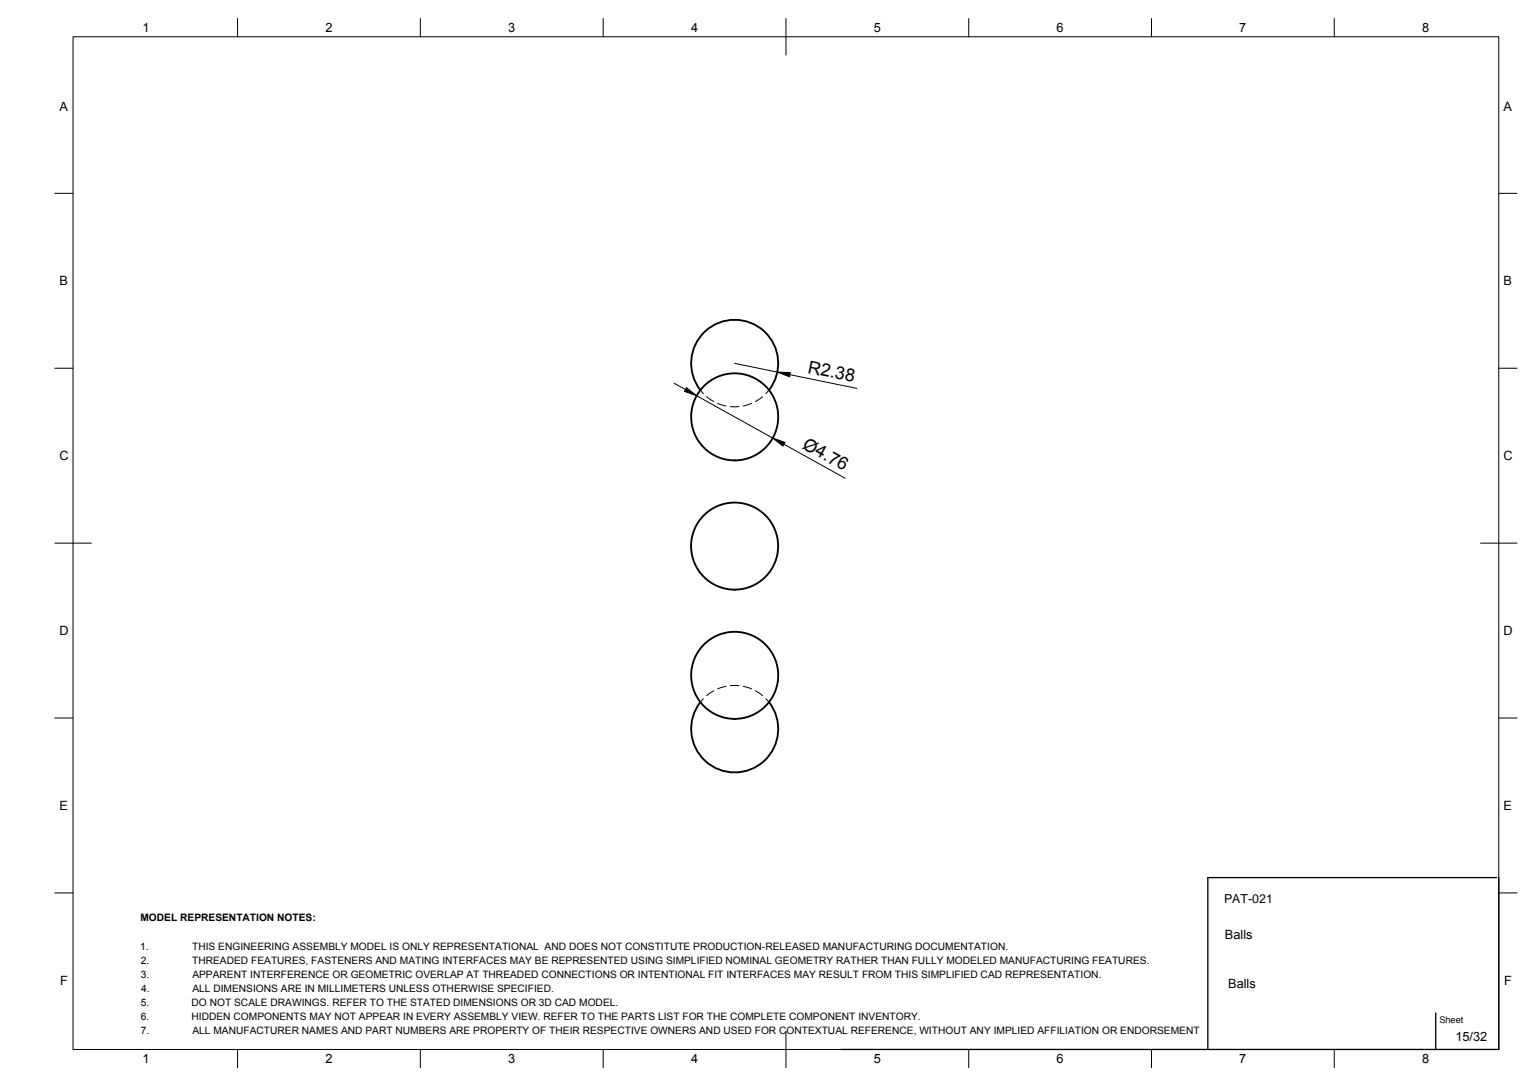
ISO-10303-21;
HEADER;
/* Generated by software containing ST-Developer
 * from STEP Tools, Inc. (www.steptools.com) 
 */

FILE_DESCRIPTION(
/* description */ ('Chain-less indexing wheel (Geneva) drive'),
/* implementation_level */ '2;1');

FILE_NAME(
/* name */ 'Balls.step',
/* time_stamp */ '2026-10-28T03:25:22-07:00',
/* author */ (''),
/* organization */ (''),
/* preprocessor_version */ 'ST-DEVELOPER v20.2',
/* originating_system */ 'Autodesk Translation Framework v15.17.0.0',
/* authorisation */ '');

FILE_SCHEMA (('AUTOMOTIVE_DESIGN { 1 0 10303 214 3 1 1 }'));
ENDSEC;

DATA;
#10=MECHANICAL_DESIGN_GEOMETRIC_PRESENTATION_REPRESENTATION('',(#312,#313,#314,#315,#316,#317,#318,#319),#10957);
#179=SPHERICAL_SURFACE('',#6312,0.23815);
#180=SPHERICAL_SURFACE('',#6314,0.23815);
#181=SPHERICAL_SURFACE('',#6316,0.23815);
#182=SPHERICAL_SURFACE('',#6318,0.23815);
#183=SPHERICAL_SURFACE('',#6320,0.23815);
#184=SPHERICAL_SURFACE('',#6322,0.23815);
#185=SPHERICAL_SURFACE('',#6324,0.23815);
#186=SPHERICAL_SURFACE('',#6326,0.23815);
#262=SHAPE_REPRESENTATION_RELATIONSHIP('SRR','None',#11076,#287);
#287=ADVANCED_BREP_SHAPE_REPRESENTATION('',(#344,#345,#346,#347,#348,#349,
#350,#351),#10939);
#312=STYLED_ITEM('',(#11287),#344);
#313=STYLED_ITEM('',(#11287),#345);
#314=STYLED_ITEM('',(#11287),#346);
#315=STYLED_ITEM('',(#11287),#347);
#316=STYLED_ITEM('',(#11287),#348);
#317=STYLED_ITEM('',(#11287),#349);
#318=STYLED_ITEM('',(#11287),#350);
#319=STYLED_ITEM('',(#11287),#351);
#344=MANIFOLD_SOLID_BREP('Body1',#5709);
#345=MANIFOLD_SOLID_BREP('Body2',#5710);
#346=MANIFOLD_SOLID_BREP('Body3',#5711);
#347=MANIFOLD_SOLID_BREP('Body4',#5712);
#348=MANIFOLD_SOLID_BREP('Body5',#5713);
#349=MANIFOLD_SOLID_BREP('Body6',#5714);
#350=MANIFOLD_SOLID_BREP('Body7',#5715);
#351=MANIFOLD_SOLID_BREP('Body8',#5716);
#793=FACE_OUTER_BOUND('',#1187,.T.);
#794=FACE_OUTER_BOUND('',#1188,.T.);
#795=FACE_OUTER_BOUND('',#1189,.T.);
#796=FACE_OUTER_BOUND('',#1190,.T.);
#797=FACE_OUTER_BOUND('',#1191,.T.);
#798=FACE_OUTER_BOUND('',#1192,.T.);
#799=FACE_OUTER_BOUND('',#1193,.T.);
#800=FACE_OUTER_BOUND('',#1194,.T.);
#1187=EDGE_LOOP('',(#4363,#4364));
#1188=EDGE_LOOP('',(#4365,#4366));
#1189=EDGE_LOOP('',(#4367,#4368));
#1190=EDGE_LOOP('',(#4369,#4370));
#1191=EDGE_LOOP('',(#4371,#4372));
#1192=EDGE_LOOP('',(#4373,#4374));
#1193=EDGE_LOOP('',(#4375,#4376));
#1194=EDGE_LOOP('',(#4377,#4378));
#2319=CIRCLE('',#6313,0.23815);
#2320=CIRCLE('',#6315,0.23815);
#2321=CIRCLE('',#6317,0.23815);
#2322=CIRCLE('',#6319,0.23815);
#2323=CIRCLE('',#6321,0.23815);
#2324=CIRCLE('',#6323,0.23815);
#2325=CIRCLE('',#6325,0.23815);
#2326=CIRCLE('',#6327,0.23815);
#2697=VERTEX_POINT('',#9322);
#2698=VERTEX_POINT('',#9323);
#2699=VERTEX_POINT('',#9326);
#2700=VERTEX_POINT('',#9327);
#2701=VERTEX_POINT('',#9330);
#2702=VERTEX_POINT('',#9331);
#2703=VERTEX_POINT('',#9334);
#2704=VERTEX_POINT('',#9335);
#2705=VERTEX_POINT('',#9338);
#2706=VERTEX_POINT('',#9339);
#2707=VERTEX_POINT('',#9342);
#2708=VERTEX_POINT('',#9343);
#2709=VERTEX_POINT('',#9346);
#2710=VERTEX_POINT('',#9347);
#2711=VERTEX_POINT('',#9350);
#2712=VERTEX_POINT('',#9351);
#3307=EDGE_CURVE('',#2697,#2698,#2319,.T.);
#3308=EDGE_CURVE('',#2699,#2700,#2320,.T.);
#3309=EDGE_CURVE('',#2701,#2702,#2321,.T.);
#3310=EDGE_CURVE('',#2703,#2704,#2322,.T.);
#3311=EDGE_CURVE('',#2705,#2706,#2323,.T.);
#3312=EDGE_CURVE('',#2707,#2708,#2324,.T.);
#3313=EDGE_CURVE('',#2709,#2710,#2325,.T.);
#3314=EDGE_CURVE('',#2711,#2712,#2326,.T.);
#4363=ORIENTED_EDGE('',*,*,#3307,.T.);
#4364=ORIENTED_EDGE('',*,*,#3307,.F.);
#4365=ORIENTED_EDGE('',*,*,#3308,.T.);
#4366=ORIENTED_EDGE('',*,*,#3308,.F.);
#4367=ORIENTED_EDGE('',*,*,#3309,.T.);
#4368=ORIENTED_EDGE('',*,*,#3309,.F.);
#4369=ORIENTED_EDGE('',*,*,#3310,.T.);
#4370=ORIENTED_EDGE('',*,*,#3310,.F.);
#4371=ORIENTED_EDGE('',*,*,#3311,.T.);
#4372=ORIENTED_EDGE('',*,*,#3311,.F.);
#4373=ORIENTED_EDGE('',*,*,#3312,.T.);
#4374=ORIENTED_EDGE('',*,*,#3312,.F.);
#4375=ORIENTED_EDGE('',*,*,#3313,.T.);
#4376=ORIENTED_EDGE('',*,*,#3313,.F.);
#4377=ORIENTED_EDGE('',*,*,#3314,.T.);
#4378=ORIENTED_EDGE('',*,*,#3314,.F.);
#5507=ADVANCED_FACE('',(#793),#179,.T.);
#5508=ADVANCED_FACE('',(#794),#180,.T.);
#5509=ADVANCED_FACE('',(#795),#181,.T.);
#5510=ADVANCED_FACE('',(#796),#182,.T.);
#5511=ADVANCED_FACE('',(#797),#183,.T.);
#5512=ADVANCED_FACE('',(#798),#184,.T.);
#5513=ADVANCED_FACE('',(#799),#185,.T.);
#5514=ADVANCED_FACE('',(#800),#186,.T.);
#5709=CLOSED_SHELL('',(#5507));
#5710=CLOSED_SHELL('',(#5508));
#5711=CLOSED_SHELL('',(#5509));
#5712=CLOSED_SHELL('',(#5510));
#5713=CLOSED_SHELL('',(#5511));
#5714=CLOSED_SHELL('',(#5512));
#5715=CLOSED_SHELL('',(#5513));
#5716=CLOSED_SHELL('',(#5514));
#6311=AXIS2_PLACEMENT_3D('',#9320,#7509,#7510);
#6312=AXIS2_PLACEMENT_3D('',#9321,#7511,#7512);
#6313=AXIS2_PLACEMENT_3D('',#9324,#7513,#7514);
#6314=AXIS2_PLACEMENT_3D('',#9325,#7515,#7516);
#6315=AXIS2_PLACEMENT_3D('',#9328,#7517,#7518);
#6316=AXIS2_PLACEMENT_3D('',#9329,#7519,#7520);
#6317=AXIS2_PLACEMENT_3D('',#9332,#7521,#7522);
#6318=AXIS2_PLACEMENT_3D('',#9333,#7523,#7524);
#6319=AXIS2_PLACEMENT_3D('',#9336,#7525,#7526);
#6320=AXIS2_PLACEMENT_3D('',#9337,#7527,#7528);
#6321=AXIS2_PLACEMENT_3D('',#9340,#7529,#7530);
#6322=AXIS2_PLACEMENT_3D('',#9341,#7531,#7532);
#6323=AXIS2_PLACEMENT_3D('',#9344,#7533,#7534);
#6324=AXIS2_PLACEMENT_3D('',#9345,#7535,#7536);
#6325=AXIS2_PLACEMENT_3D('',#9348,#7537,#7538);
#6326=AXIS2_PLACEMENT_3D('',#9349,#7539,#7540);
#6327=AXIS2_PLACEMENT_3D('',#9352,#7541,#7542);
#7509=DIRECTION('axis',(0.,0.,1.));
#7510=DIRECTION('refdir',(1.,0.,0.));
#7511=DIRECTION('center_axis',(0.,0.,1.));
#7512=DIRECTION('ref_axis',(1.,0.,0.));
#7513=DIRECTION('center_axis',(1.22464679914735E-16,-1.,0.));
#7514=DIRECTION('ref_axis',(-1.,-1.22464679914735E-16,0.));
#7515=DIRECTION('center_axis',(0.707106781186548,0.,0.707106781186548));
#7516=DIRECTION('ref_axis',(0.707106781186548,0.,-0.707106781186548));
#7517=DIRECTION('center_axis',(8.65956056235494E-17,-1.,-8.65956056235493E-17));
#7518=DIRECTION('ref_axis',(-0.707106781186547,-1.22464679914735E-16,0.707106781186547));
#7519=DIRECTION('center_axis',(1.,0.,0.));
#7520=DIRECTION('ref_axis',(6.12323399573676E-17,0.,-1.));
#7521=DIRECTION('center_axis',(7.49879891330929E-33,-1.,-1.22464679914735E-16));
#7522=DIRECTION('ref_axis',(-6.12323399573676E-17,-1.22464679914735E-16,
1.));
#7523=DIRECTION('center_axis',(0.707106781186548,0.,-0.707106781186548));
#7524=DIRECTION('ref_axis',(-0.707106781186548,0.,-0.707106781186548));
#7525=DIRECTION('center_axis',(-8.65956056235493E-17,-1.,-8.65956056235494E-17));
#7526=DIRECTION('ref_axis',(0.707106781186547,-1.22464679914735E-16,0.707106781186547));
#7527=DIRECTION('center_axis',(0.,0.,-1.));
#7528=DIRECTION('ref_axis',(-1.,0.,-1.22464679914735E-16));
#7529=DIRECTION('center_axis',(-1.22464679914735E-16,-1.,-1.49975978266186E-32));
#7530=DIRECTION('ref_axis',(1.,-1.22464679914735E-16,1.22464679914735E-16));
#7531=DIRECTION('center_axis',(-0.707106781186547,0.,-0.707106781186548));
#7532=DIRECTION('ref_axis',(-0.707106781186548,0.,0.707106781186547));
#7533=DIRECTION('center_axis',(-8.65956056235493E-17,-1.,8.65956056235493E-17));
#7534=DIRECTION('ref_axis',(0.707106781186548,-1.22464679914735E-16,-0.707106781186547));
#7535=DIRECTION('center_axis',(-1.,0.,0.));
#7536=DIRECTION('ref_axis',(-1.83697019872103E-16,0.,1.));
#7537=DIRECTION('center_axis',(-2.24963967399279E-32,-1.,1.22464679914735E-16));
#7538=DIRECTION('ref_axis',(1.83697019872103E-16,-1.22464679914735E-16,
-1.));
#7539=DIRECTION('center_axis',(-0.707106781186548,0.,0.707106781186548));
#7540=DIRECTION('ref_axis',(0.707106781186547,0.,0.707106781186548));
#7541=DIRECTION('center_axis',(8.65956056235493E-17,-1.,8.65956056235493E-17));
#7542=DIRECTION('ref_axis',(-0.707106781186547,-1.22464679914735E-16,-0.707106781186548));
#9320=CARTESIAN_POINT('',(0.,0.,0.));
#9321=CARTESIAN_POINT('Origin',(1.,0.,0.));
#9322=CARTESIAN_POINT('',(1.,-1.78583896120461E-33,0.23815));
#9323=CARTESIAN_POINT('',(1.,-1.78583896120461E-33,-0.23815));
#9324=CARTESIAN_POINT('Origin',(1.,0.,0.));
#9325=CARTESIAN_POINT('Origin',(0.707106781186548,0.,-0.707106781186547));
#9326=CARTESIAN_POINT('',(0.875504261126124,-1.78583896120461E-33,-0.538709301246971));
#9327=CARTESIAN_POINT('',(0.538709301246971,-1.78583896120461E-33,-0.875504261126124));
#9328=CARTESIAN_POINT('Origin',(0.707106781186548,0.,-0.707106781186547));
#9329=CARTESIAN_POINT('Origin',(6.12323399573677E-17,0.,-1.));
#9330=CARTESIAN_POINT('',(0.23815,-1.78583896120461E-33,-1.));
#9331=CARTESIAN_POINT('',(-0.23815,-1.78583896120461E-33,-1.));
#9332=CARTESIAN_POINT('Origin',(6.12323399573677E-17,0.,-1.));
#9333=CARTESIAN_POINT('Origin',(-0.707106781186547,0.,-0.707106781186548));
#9334=CARTESIAN_POINT('',(-0.538709301246971,-1.78583896120461E-33,-0.875504261126124));
#9335=CARTESIAN_POINT('',(-0.875504261126124,-1.78583896120461E-33,-0.538709301246971));
#9336=CARTESIAN_POINT('Origin',(-0.707106781186547,0.,-0.707106781186548));
#9337=CARTESIAN_POINT('Origin',(-1.,0.,-1.22464679914735E-16));
#9338=CARTESIAN_POINT('',(-1.,-1.78583896120461E-33,-0.23815));
#9339=CARTESIAN_POINT('',(-1.,-1.78583896120461E-33,0.23815));
#9340=CARTESIAN_POINT('Origin',(-1.,0.,-1.22464679914735E-16));
#9341=CARTESIAN_POINT('Origin',(-0.707106781186548,0.,0.707106781186547));
#9342=CARTESIAN_POINT('',(-0.875504261126124,-7.94881478324376E-33,0.538709301246971));
#9343=CARTESIAN_POINT('',(-0.538709301246971,4.37713686083455E-33,0.875504261126124));
#9344=CARTESIAN_POINT('Origin',(-0.707106781186548,0.,0.707106781186547));
#9345=CARTESIAN_POINT('Origin',(-1.83697019872103E-16,0.,1.));
#9346=CARTESIAN_POINT('',(-0.23815,-1.78583896120461E-33,1.));
#9347=CARTESIAN_POINT('',(0.23815,-1.78583896120461E-33,1.));
#9348=CARTESIAN_POINT('Origin',(-1.83697019872103E-16,0.,1.));
#9349=CARTESIAN_POINT('Origin',(0.707106781186547,0.,0.707106781186548));
#9350=CARTESIAN_POINT('',(0.538709301246971,-4.86732687222419E-33,0.875504261126124));
#9351=CARTESIAN_POINT('',(0.875504261126124,1.29564894981497E-33,0.538709301246971));
#9352=CARTESIAN_POINT('Origin',(0.707106781186547,0.,0.707106781186548));
#10908=UNCERTAINTY_MEASURE_WITH_UNIT(LENGTH_MEASURE(0.001),#10958,
'DISTANCE_ACCURACY_VALUE',
'Maximum model space distance between geometric entities at asserted c
onnectivities');
#10926=UNCERTAINTY_MEASURE_WITH_UNIT(LENGTH_MEASURE(0.001),#10958,
'DISTANCE_ACCURACY_VALUE',
'Maximum model space distance between geometric entities at asserted c
onnectivities');
#10939=(
GEOMETRIC_REPRESENTATION_CONTEXT(3)
GLOBAL_UNCERTAINTY_ASSIGNED_CONTEXT((#10908))
GLOBAL_UNIT_ASSIGNED_CONTEXT((#10958,#10960,#10961))
REPRESENTATION_CONTEXT('','3D')
);
#10957=(
GEOMETRIC_REPRESENTATION_CONTEXT(3)
GLOBAL_UNCERTAINTY_ASSIGNED_CONTEXT((#10926))
GLOBAL_UNIT_ASSIGNED_CONTEXT((#10958,#10960,#10961))
REPRESENTATION_CONTEXT('','3D')
);
#10958=(
LENGTH_UNIT()
NAMED_UNIT(*)
SI_UNIT(.CENTI.,.METRE.)
);
#10960=(
NAMED_UNIT(*)
PLANE_ANGLE_UNIT()
SI_UNIT($,.RADIAN.)
);
#10961=(
NAMED_UNIT(*)
SI_UNIT($,.STERADIAN.)
SOLID_ANGLE_UNIT()
);
#10974=SHAPE_DEFINITION_REPRESENTATION(#11004,#11076);
#11004=PRODUCT_DEFINITION_SHAPE('',$,#11107);
#11076=SHAPE_REPRESENTATION('',(#6311),#10939);
#11094=PRODUCT_DEFINITION_CONTEXT('part definition',#11186,'design');
#11107=PRODUCT_DEFINITION('Balls','Balls',#11137,#11094);
#11137=PRODUCT_DEFINITION_FORMATION('',$,#11200);
#11186=APPLICATION_CONTEXT(
'Core Data for Automotive Mechanical Design Process');
#11187=PRODUCT_CONTEXT('part definition',#11186,'mechanical');
#11200=PRODUCT('Balls','Balls','Balls',(#11187));
#11281=COLOUR_RGB('Grey',0.48,0.52,0.57);
#11282=FILL_AREA_STYLE_COLOUR('',#11281);
#11283=FILL_AREA_STYLE('',(#11282));
#11284=SURFACE_STYLE_FILL_AREA(#11283);
#11285=SURFACE_SIDE_STYLE('',(#11284));
#11286=SURFACE_STYLE_USAGE(.BOTH.,#11285);
#11287=PRESENTATION_STYLE_ASSIGNMENT((#11286));
ENDSEC;
END-ISO-10303-21;
